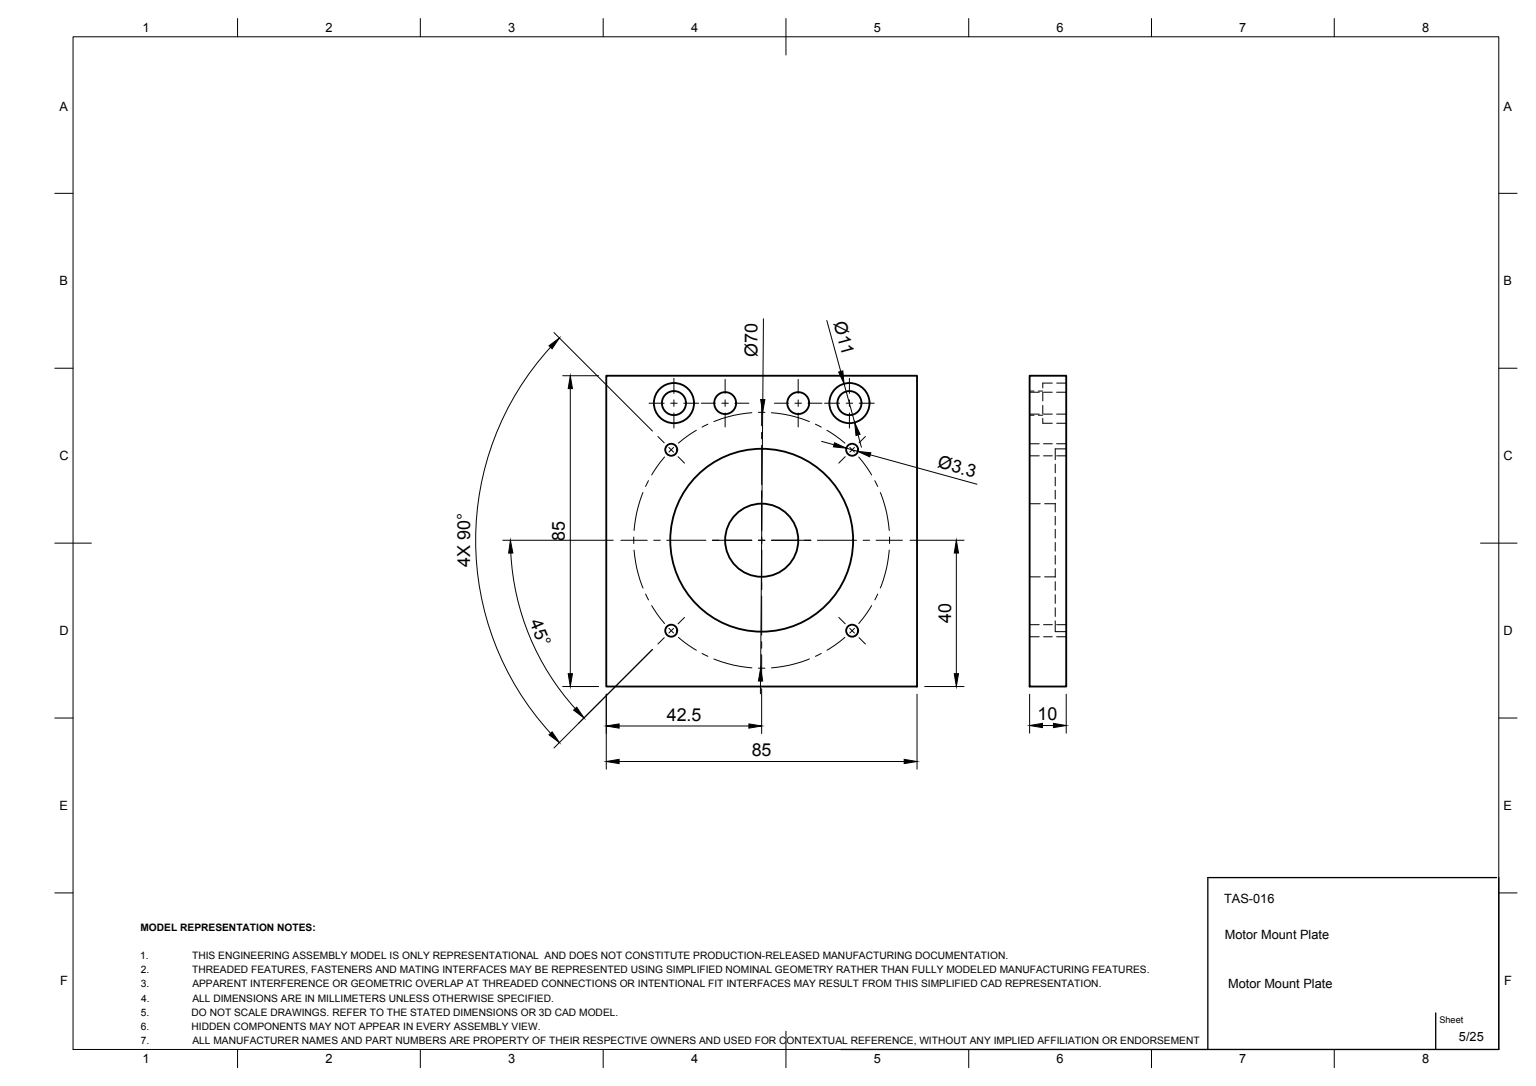
ISO-10303-21;
HEADER;
/* Generated by software containing ST-Developer
 * from STEP Tools, Inc. (www.steptools.com) 
 */

FILE_DESCRIPTION(
/* description */ ('STEP AP214'),
/* implementation_level */ '2;1');

FILE_NAME(
/* name */ 'Motor Mount Plate.step',
/* time_stamp */ '2026-11-15T14:55:55-08:00',
/* author */ (''),
/* organization */ (''),
/* preprocessor_version */ 'ST-DEVELOPER v20.2',
/* originating_system */ 'Autodesk Translation Framework v15.17.0.0',
/* authorisation */ '');

FILE_SCHEMA (('AUTOMOTIVE_DESIGN { 1 0 10303 214 3 1 1 }'));
ENDSEC;

DATA;
#10=MECHANICAL_DESIGN_GEOMETRIC_PRESENTATION_REPRESENTATION('',(#938),#57079);
#878=SHAPE_REPRESENTATION_RELATIONSHIP('SRR','None',#57264,#907);
#907=ADVANCED_BREP_SHAPE_REPRESENTATION('',(#975),#57056);
#938=STYLED_ITEM('',(#57444),#975);
#975=MANIFOLD_SOLID_BREP('Body1',#24538);
#1109=FACE_BOUND('',#3951,.T.);
#1110=FACE_BOUND('',#3952,.T.);
#1111=FACE_BOUND('',#3953,.T.);
#1112=FACE_BOUND('',#3954,.T.);
#1113=FACE_BOUND('',#3955,.T.);
#1114=FACE_BOUND('',#3956,.T.);
#1115=FACE_BOUND('',#3957,.T.);
#1116=FACE_BOUND('',#3958,.T.);
#1117=FACE_BOUND('',#3959,.T.);
#1118=FACE_BOUND('',#3965,.T.);
#1119=FACE_BOUND('',#3966,.T.);
#1120=FACE_BOUND('',#3967,.T.);
#1121=FACE_BOUND('',#3968,.T.);
#1122=FACE_BOUND('',#3969,.T.);
#1123=FACE_BOUND('',#3970,.T.);
#1124=FACE_BOUND('',#3971,.T.);
#1125=FACE_BOUND('',#3972,.T.);
#1126=FACE_BOUND('',#3973,.T.);
#1127=FACE_BOUND('',#3975,.T.);
#1128=FACE_BOUND('',#3977,.T.);
#1129=FACE_BOUND('',#3979,.T.);
#1524=PLANE('',#25459);
#1525=PLANE('',#25460);
#1526=PLANE('',#25461);
#1527=PLANE('',#25462);
#1528=PLANE('',#25463);
#1529=PLANE('',#25464);
#1530=PLANE('',#25465);
#1531=PLANE('',#25466);
#1532=PLANE('',#25467);
#2454=FACE_OUTER_BOUND('',#3938,.T.);
#2455=FACE_OUTER_BOUND('',#3939,.T.);
#2456=FACE_OUTER_BOUND('',#3940,.T.);
#2457=FACE_OUTER_BOUND('',#3941,.T.);
#2458=FACE_OUTER_BOUND('',#3942,.T.);
#2459=FACE_OUTER_BOUND('',#3943,.T.);
#2460=FACE_OUTER_BOUND('',#3944,.T.);
#2461=FACE_OUTER_BOUND('',#3945,.T.);
#2462=FACE_OUTER_BOUND('',#3946,.T.);
#2463=FACE_OUTER_BOUND('',#3947,.T.);
#2464=FACE_OUTER_BOUND('',#3948,.T.);
#2465=FACE_OUTER_BOUND('',#3949,.T.);
#2466=FACE_OUTER_BOUND('',#3950,.T.);
#2467=FACE_OUTER_BOUND('',#3960,.T.);
#2468=FACE_OUTER_BOUND('',#3961,.T.);
#2469=FACE_OUTER_BOUND('',#3962,.T.);
#2470=FACE_OUTER_BOUND('',#3963,.T.);
#2471=FACE_OUTER_BOUND('',#3964,.T.);
#2472=FACE_OUTER_BOUND('',#3974,.T.);
#2473=FACE_OUTER_BOUND('',#3976,.T.);
#2474=FACE_OUTER_BOUND('',#3978,.T.);
#3938=EDGE_LOOP('',(#17264,#17265,#17266,#17267));
#3939=EDGE_LOOP('',(#17268,#17269,#17270,#17271));
#3940=EDGE_LOOP('',(#17272,#17273,#17274,#17275));
#3941=EDGE_LOOP('',(#17276,#17277,#17278,#17279));
#3942=EDGE_LOOP('',(#17280,#17281,#17282,#17283));
#3943=EDGE_LOOP('',(#17284,#17285,#17286,#17287));
#3944=EDGE_LOOP('',(#17288,#17289,#17290,#17291));
#3945=EDGE_LOOP('',(#17292,#17293,#17294,#17295));
#3946=EDGE_LOOP('',(#17296,#17297,#17298,#17299));
#3947=EDGE_LOOP('',(#17300,#17301,#17302,#17303));
#3948=EDGE_LOOP('',(#17304,#17305,#17306,#17307));
#3949=EDGE_LOOP('',(#17308,#17309,#17310,#17311));
#3950=EDGE_LOOP('',(#17312,#17313,#17314,#17315));
#3951=EDGE_LOOP('',(#17316));
#3952=EDGE_LOOP('',(#17317));
#3953=EDGE_LOOP('',(#17318));
#3954=EDGE_LOOP('',(#17319));
#3955=EDGE_LOOP('',(#17320));
#3956=EDGE_LOOP('',(#17321));
#3957=EDGE_LOOP('',(#17322));
#3958=EDGE_LOOP('',(#17323));
#3959=EDGE_LOOP('',(#17324));
#3960=EDGE_LOOP('',(#17325,#17326,#17327,#17328));
#3961=EDGE_LOOP('',(#17329,#17330,#17331,#17332));
#3962=EDGE_LOOP('',(#17333,#17334,#17335,#17336));
#3963=EDGE_LOOP('',(#17337,#17338,#17339,#17340));
#3964=EDGE_LOOP('',(#17341,#17342,#17343,#17344));
#3965=EDGE_LOOP('',(#17345));
#3966=EDGE_LOOP('',(#17346));
#3967=EDGE_LOOP('',(#17347));
#3968=EDGE_LOOP('',(#17348));
#3969=EDGE_LOOP('',(#17349));
#3970=EDGE_LOOP('',(#17350));
#3971=EDGE_LOOP('',(#17351));
#3972=EDGE_LOOP('',(#17352));
#3973=EDGE_LOOP('',(#17353));
#3974=EDGE_LOOP('',(#17354));
#3975=EDGE_LOOP('',(#17355));
#3976=EDGE_LOOP('',(#17356));
#3977=EDGE_LOOP('',(#17357));
#3978=EDGE_LOOP('',(#17358));
#3979=EDGE_LOOP('',(#17359));
#5689=LINE('',#36296,#7656);
#5690=LINE('',#36302,#7657);
#5691=LINE('',#36308,#7658);
#5692=LINE('',#36314,#7659);
#5693=LINE('',#36320,#7660);
#5694=LINE('',#36326,#7661);
#5695=LINE('',#36332,#7662);
#5696=LINE('',#36338,#7663);
#5697=LINE('',#36344,#7664);
#5698=LINE('',#36350,#7665);
#5699=LINE('',#36356,#7666);
#5700=LINE('',#36362,#7667);
#5701=LINE('',#36367,#7668);
#5702=LINE('',#36369,#7669);
#5703=LINE('',#36371,#7670);
#5704=LINE('',#36372,#7671);
#5705=LINE('',#36376,#7672);
#5706=LINE('',#36377,#7673);
#5707=LINE('',#36378,#7674);
#5708=LINE('',#36381,#7675);
#5709=LINE('',#36382,#7676);
#5710=LINE('',#36385,#7677);
#5711=LINE('',#36386,#7678);
#5712=LINE('',#36388,#7679);
#7656=VECTOR('',#28999,1.65);
#7657=VECTOR('',#29006,1.65);
#7658=VECTOR('',#29013,1.65);
#7659=VECTOR('',#29020,1.65);
#7660=VECTOR('',#29027,3.);
#7661=VECTOR('',#29034,3.);
#7662=VECTOR('',#29041,5.5);
#7663=VECTOR('',#29048,3.3);
#7664=VECTOR('',#29055,5.5);
#7665=VECTOR('',#29062,3.3);
#7666=VECTOR('',#29069,10.);
#7667=VECTOR('',#29076,25.);
#7668=VECTOR('',#29081,1000.);
#7669=VECTOR('',#29082,1000.);
#7670=VECTOR('',#29083,1000.);
#7671=VECTOR('',#29084,1000.);
#7672=VECTOR('',#29087,1000.);
#7673=VECTOR('',#29088,1000.);
#7674=VECTOR('',#29089,1000.);
#7675=VECTOR('',#29092,1000.);
#7676=VECTOR('',#29093,1000.);
#7677=VECTOR('',#29096,1000.);
#7678=VECTOR('',#29097,1000.);
#7679=VECTOR('',#29100,1000.);
#9406=CIRCLE('',#25424,1.65);
#9407=CIRCLE('',#25425,1.65);
#9408=CIRCLE('',#25427,1.65);
#9409=CIRCLE('',#25428,1.65);
#9410=CIRCLE('',#25430,1.65);
#9411=CIRCLE('',#25431,1.65);
#9412=CIRCLE('',#25433,1.65);
#9413=CIRCLE('',#25434,1.65);
#9414=CIRCLE('',#25436,3.);
#9415=CIRCLE('',#25437,3.);
#9416=CIRCLE('',#25439,3.);
#9417=CIRCLE('',#25440,3.);
#9418=CIRCLE('',#25442,5.5);
#9419=CIRCLE('',#25443,5.5);
#9420=CIRCLE('',#25445,3.3);
#9421=CIRCLE('',#25446,3.3);
#9422=CIRCLE('',#25448,5.5);
#9423=CIRCLE('',#25449,5.5);
#9424=CIRCLE('',#25451,3.3);
#9425=CIRCLE('',#25452,3.3);
#9426=CIRCLE('',#25454,10.);
#9427=CIRCLE('',#25455,10.);
#9428=CIRCLE('',#25457,25.);
#9429=CIRCLE('',#25458,25.);
#10719=VERTEX_POINT('',#36293);
#10720=VERTEX_POINT('',#36295);
#10721=VERTEX_POINT('',#36299);
#10722=VERTEX_POINT('',#36301);
#10723=VERTEX_POINT('',#36305);
#10724=VERTEX_POINT('',#36307);
#10725=VERTEX_POINT('',#36311);
#10726=VERTEX_POINT('',#36313);
#10727=VERTEX_POINT('',#36317);
#10728=VERTEX_POINT('',#36319);
#10729=VERTEX_POINT('',#36323);
#10730=VERTEX_POINT('',#36325);
#10731=VERTEX_POINT('',#36329);
#10732=VERTEX_POINT('',#36331);
#10733=VERTEX_POINT('',#36335);
#10734=VERTEX_POINT('',#36337);
#10735=VERTEX_POINT('',#36341);
#10736=VERTEX_POINT('',#36343);
#10737=VERTEX_POINT('',#36347);
#10738=VERTEX_POINT('',#36349);
#10739=VERTEX_POINT('',#36353);
#10740=VERTEX_POINT('',#36355);
#10741=VERTEX_POINT('',#36359);
#10742=VERTEX_POINT('',#36361);
#10743=VERTEX_POINT('',#36365);
#10744=VERTEX_POINT('',#36366);
#10745=VERTEX_POINT('',#36368);
#10746=VERTEX_POINT('',#36370);
#10747=VERTEX_POINT('',#36374);
#10748=VERTEX_POINT('',#36375);
#10749=VERTEX_POINT('',#36380);
#10750=VERTEX_POINT('',#36384);
#13177=EDGE_CURVE('',#10719,#10719,#9406,.T.);
#13178=EDGE_CURVE('',#10719,#10720,#5689,.T.);
#13179=EDGE_CURVE('',#10720,#10720,#9407,.T.);
#13180=EDGE_CURVE('',#10721,#10721,#9408,.T.);
#13181=EDGE_CURVE('',#10721,#10722,#5690,.T.);
#13182=EDGE_CURVE('',#10722,#10722,#9409,.T.);
#13183=EDGE_CURVE('',#10723,#10723,#9410,.T.);
#13184=EDGE_CURVE('',#10723,#10724,#5691,.T.);
#13185=EDGE_CURVE('',#10724,#10724,#9411,.T.);
#13186=EDGE_CURVE('',#10725,#10725,#9412,.T.);
#13187=EDGE_CURVE('',#10725,#10726,#5692,.T.);
#13188=EDGE_CURVE('',#10726,#10726,#9413,.T.);
#13189=EDGE_CURVE('',#10727,#10727,#9414,.T.);
#13190=EDGE_CURVE('',#10727,#10728,#5693,.T.);
#13191=EDGE_CURVE('',#10728,#10728,#9415,.T.);
#13192=EDGE_CURVE('',#10729,#10729,#9416,.T.);
#13193=EDGE_CURVE('',#10729,#10730,#5694,.T.);
#13194=EDGE_CURVE('',#10730,#10730,#9417,.T.);
#13195=EDGE_CURVE('',#10731,#10731,#9418,.T.);
#13196=EDGE_CURVE('',#10731,#10732,#5695,.T.);
#13197=EDGE_CURVE('',#10732,#10732,#9419,.T.);
#13198=EDGE_CURVE('',#10733,#10733,#9420,.T.);
#13199=EDGE_CURVE('',#10733,#10734,#5696,.T.);
#13200=EDGE_CURVE('',#10734,#10734,#9421,.T.);
#13201=EDGE_CURVE('',#10735,#10735,#9422,.T.);
#13202=EDGE_CURVE('',#10735,#10736,#5697,.T.);
#13203=EDGE_CURVE('',#10736,#10736,#9423,.T.);
#13204=EDGE_CURVE('',#10737,#10737,#9424,.T.);
#13205=EDGE_CURVE('',#10737,#10738,#5698,.T.);
#13206=EDGE_CURVE('',#10738,#10738,#9425,.T.);
#13207=EDGE_CURVE('',#10739,#10739,#9426,.T.);
#13208=EDGE_CURVE('',#10739,#10740,#5699,.T.);
#13209=EDGE_CURVE('',#10740,#10740,#9427,.T.);
#13210=EDGE_CURVE('',#10741,#10741,#9428,.T.);
#13211=EDGE_CURVE('',#10741,#10742,#5700,.T.);
#13212=EDGE_CURVE('',#10742,#10742,#9429,.T.);
#13213=EDGE_CURVE('',#10743,#10744,#5701,.T.);
#13214=EDGE_CURVE('',#10744,#10745,#5702,.T.);
#13215=EDGE_CURVE('',#10745,#10746,#5703,.T.);
#13216=EDGE_CURVE('',#10746,#10743,#5704,.T.);
#13217=EDGE_CURVE('',#10747,#10748,#5705,.T.);
#13218=EDGE_CURVE('',#10744,#10748,#5706,.T.);
#13219=EDGE_CURVE('',#10743,#10747,#5707,.T.);
#13220=EDGE_CURVE('',#10748,#10749,#5708,.T.);
#13221=EDGE_CURVE('',#10745,#10749,#5709,.T.);
#13222=EDGE_CURVE('',#10749,#10750,#5710,.T.);
#13223=EDGE_CURVE('',#10746,#10750,#5711,.T.);
#13224=EDGE_CURVE('',#10750,#10747,#5712,.T.);
#17264=ORIENTED_EDGE('',*,*,#13177,.F.);
#17265=ORIENTED_EDGE('',*,*,#13178,.T.);
#17266=ORIENTED_EDGE('',*,*,#13179,.T.);
#17267=ORIENTED_EDGE('',*,*,#13178,.F.);
#17268=ORIENTED_EDGE('',*,*,#13180,.F.);
#17269=ORIENTED_EDGE('',*,*,#13181,.T.);
#17270=ORIENTED_EDGE('',*,*,#13182,.T.);
#17271=ORIENTED_EDGE('',*,*,#13181,.F.);
#17272=ORIENTED_EDGE('',*,*,#13183,.F.);
#17273=ORIENTED_EDGE('',*,*,#13184,.T.);
#17274=ORIENTED_EDGE('',*,*,#13185,.T.);
#17275=ORIENTED_EDGE('',*,*,#13184,.F.);
#17276=ORIENTED_EDGE('',*,*,#13186,.F.);
#17277=ORIENTED_EDGE('',*,*,#13187,.T.);
#17278=ORIENTED_EDGE('',*,*,#13188,.T.);
#17279=ORIENTED_EDGE('',*,*,#13187,.F.);
#17280=ORIENTED_EDGE('',*,*,#13189,.F.);
#17281=ORIENTED_EDGE('',*,*,#13190,.T.);
#17282=ORIENTED_EDGE('',*,*,#13191,.T.);
#17283=ORIENTED_EDGE('',*,*,#13190,.F.);
#17284=ORIENTED_EDGE('',*,*,#13192,.F.);
#17285=ORIENTED_EDGE('',*,*,#13193,.T.);
#17286=ORIENTED_EDGE('',*,*,#13194,.T.);
#17287=ORIENTED_EDGE('',*,*,#13193,.F.);
#17288=ORIENTED_EDGE('',*,*,#13195,.F.);
#17289=ORIENTED_EDGE('',*,*,#13196,.T.);
#17290=ORIENTED_EDGE('',*,*,#13197,.T.);
#17291=ORIENTED_EDGE('',*,*,#13196,.F.);
#17292=ORIENTED_EDGE('',*,*,#13198,.F.);
#17293=ORIENTED_EDGE('',*,*,#13199,.T.);
#17294=ORIENTED_EDGE('',*,*,#13200,.T.);
#17295=ORIENTED_EDGE('',*,*,#13199,.F.);
#17296=ORIENTED_EDGE('',*,*,#13201,.F.);
#17297=ORIENTED_EDGE('',*,*,#13202,.T.);
#17298=ORIENTED_EDGE('',*,*,#13203,.T.);
#17299=ORIENTED_EDGE('',*,*,#13202,.F.);
#17300=ORIENTED_EDGE('',*,*,#13204,.F.);
#17301=ORIENTED_EDGE('',*,*,#13205,.T.);
#17302=ORIENTED_EDGE('',*,*,#13206,.T.);
#17303=ORIENTED_EDGE('',*,*,#13205,.F.);
#17304=ORIENTED_EDGE('',*,*,#13207,.F.);
#17305=ORIENTED_EDGE('',*,*,#13208,.T.);
#17306=ORIENTED_EDGE('',*,*,#13209,.T.);
#17307=ORIENTED_EDGE('',*,*,#13208,.F.);
#17308=ORIENTED_EDGE('',*,*,#13210,.F.);
#17309=ORIENTED_EDGE('',*,*,#13211,.T.);
#17310=ORIENTED_EDGE('',*,*,#13212,.T.);
#17311=ORIENTED_EDGE('',*,*,#13211,.F.);
#17312=ORIENTED_EDGE('',*,*,#13213,.T.);
#17313=ORIENTED_EDGE('',*,*,#13214,.T.);
#17314=ORIENTED_EDGE('',*,*,#13215,.T.);
#17315=ORIENTED_EDGE('',*,*,#13216,.T.);
#17316=ORIENTED_EDGE('',*,*,#13185,.F.);
#17317=ORIENTED_EDGE('',*,*,#13179,.F.);
#17318=ORIENTED_EDGE('',*,*,#13182,.F.);
#17319=ORIENTED_EDGE('',*,*,#13188,.F.);
#17320=ORIENTED_EDGE('',*,*,#13191,.F.);
#17321=ORIENTED_EDGE('',*,*,#13194,.F.);
#17322=ORIENTED_EDGE('',*,*,#13197,.F.);
#17323=ORIENTED_EDGE('',*,*,#13203,.F.);
#17324=ORIENTED_EDGE('',*,*,#13212,.F.);
#17325=ORIENTED_EDGE('',*,*,#13217,.T.);
#17326=ORIENTED_EDGE('',*,*,#13218,.F.);
#17327=ORIENTED_EDGE('',*,*,#13213,.F.);
#17328=ORIENTED_EDGE('',*,*,#13219,.T.);
#17329=ORIENTED_EDGE('',*,*,#13220,.T.);
#17330=ORIENTED_EDGE('',*,*,#13221,.F.);
#17331=ORIENTED_EDGE('',*,*,#13214,.F.);
#17332=ORIENTED_EDGE('',*,*,#13218,.T.);
#17333=ORIENTED_EDGE('',*,*,#13222,.T.);
#17334=ORIENTED_EDGE('',*,*,#13223,.F.);
#17335=ORIENTED_EDGE('',*,*,#13215,.F.);
#17336=ORIENTED_EDGE('',*,*,#13221,.T.);
#17337=ORIENTED_EDGE('',*,*,#13224,.T.);
#17338=ORIENTED_EDGE('',*,*,#13219,.F.);
#17339=ORIENTED_EDGE('',*,*,#13216,.F.);
#17340=ORIENTED_EDGE('',*,*,#13223,.T.);
#17341=ORIENTED_EDGE('',*,*,#13217,.F.);
#17342=ORIENTED_EDGE('',*,*,#13224,.F.);
#17343=ORIENTED_EDGE('',*,*,#13222,.F.);
#17344=ORIENTED_EDGE('',*,*,#13220,.F.);
#17345=ORIENTED_EDGE('',*,*,#13177,.T.);
#17346=ORIENTED_EDGE('',*,*,#13180,.T.);
#17347=ORIENTED_EDGE('',*,*,#13183,.T.);
#17348=ORIENTED_EDGE('',*,*,#13186,.T.);
#17349=ORIENTED_EDGE('',*,*,#13189,.T.);
#17350=ORIENTED_EDGE('',*,*,#13192,.T.);
#17351=ORIENTED_EDGE('',*,*,#13198,.T.);
#17352=ORIENTED_EDGE('',*,*,#13204,.T.);
#17353=ORIENTED_EDGE('',*,*,#13207,.T.);
#17354=ORIENTED_EDGE('',*,*,#13210,.T.);
#17355=ORIENTED_EDGE('',*,*,#13209,.F.);
#17356=ORIENTED_EDGE('',*,*,#13201,.T.);
#17357=ORIENTED_EDGE('',*,*,#13206,.F.);
#17358=ORIENTED_EDGE('',*,*,#13195,.T.);
#17359=ORIENTED_EDGE('',*,*,#13200,.F.);
#22826=CYLINDRICAL_SURFACE('',#25423,1.65);
#22827=CYLINDRICAL_SURFACE('',#25426,1.65);
#22828=CYLINDRICAL_SURFACE('',#25429,1.65);
#22829=CYLINDRICAL_SURFACE('',#25432,1.65);
#22830=CYLINDRICAL_SURFACE('',#25435,3.);
#22831=CYLINDRICAL_SURFACE('',#25438,3.);
#22832=CYLINDRICAL_SURFACE('',#25441,5.5);
#22833=CYLINDRICAL_SURFACE('',#25444,3.3);
#22834=CYLINDRICAL_SURFACE('',#25447,5.5);
#22835=CYLINDRICAL_SURFACE('',#25450,3.3);
#22836=CYLINDRICAL_SURFACE('',#25453,10.);
#22837=CYLINDRICAL_SURFACE('',#25456,25.);
#23446=ADVANCED_FACE('',(#2454),#22826,.F.);
#23447=ADVANCED_FACE('',(#2455),#22827,.F.);
#23448=ADVANCED_FACE('',(#2456),#22828,.F.);
#23449=ADVANCED_FACE('',(#2457),#22829,.F.);
#23450=ADVANCED_FACE('',(#2458),#22830,.F.);
#23451=ADVANCED_FACE('',(#2459),#22831,.F.);
#23452=ADVANCED_FACE('',(#2460),#22832,.F.);
#23453=ADVANCED_FACE('',(#2461),#22833,.F.);
#23454=ADVANCED_FACE('',(#2462),#22834,.F.);
#23455=ADVANCED_FACE('',(#2463),#22835,.F.);
#23456=ADVANCED_FACE('',(#2464),#22836,.F.);
#23457=ADVANCED_FACE('',(#2465),#22837,.F.);
#23458=ADVANCED_FACE('',(#2466,#1109,#1110,#1111,#1112,#1113,#1114,#1115,
#1116,#1117),#1524,.F.);
#23459=ADVANCED_FACE('',(#2467),#1525,.F.);
#23460=ADVANCED_FACE('',(#2468),#1526,.F.);
#23461=ADVANCED_FACE('',(#2469),#1527,.F.);
#23462=ADVANCED_FACE('',(#2470),#1528,.F.);
#23463=ADVANCED_FACE('',(#2471,#1118,#1119,#1120,#1121,#1122,#1123,#1124,
#1125,#1126),#1529,.T.);
#23464=ADVANCED_FACE('',(#2472,#1127),#1530,.T.);
#23465=ADVANCED_FACE('',(#2473,#1128),#1531,.F.);
#23466=ADVANCED_FACE('',(#2474,#1129),#1532,.F.);
#24538=CLOSED_SHELL('',(#23446,#23447,#23448,#23449,#23450,#23451,#23452,
#23453,#23454,#23455,#23456,#23457,#23458,#23459,#23460,#23461,#23462,#23463,
#23464,#23465,#23466));
#25422=AXIS2_PLACEMENT_3D('',#36291,#28993,#28994);
#25423=AXIS2_PLACEMENT_3D('',#36292,#28995,#28996);
#25424=AXIS2_PLACEMENT_3D('',#36294,#28997,#28998);
#25425=AXIS2_PLACEMENT_3D('',#36297,#29000,#29001);
#25426=AXIS2_PLACEMENT_3D('',#36298,#29002,#29003);
#25427=AXIS2_PLACEMENT_3D('',#36300,#29004,#29005);
#25428=AXIS2_PLACEMENT_3D('',#36303,#29007,#29008);
#25429=AXIS2_PLACEMENT_3D('',#36304,#29009,#29010);
#25430=AXIS2_PLACEMENT_3D('',#36306,#29011,#29012);
#25431=AXIS2_PLACEMENT_3D('',#36309,#29014,#29015);
#25432=AXIS2_PLACEMENT_3D('',#36310,#29016,#29017);
#25433=AXIS2_PLACEMENT_3D('',#36312,#29018,#29019);
#25434=AXIS2_PLACEMENT_3D('',#36315,#29021,#29022);
#25435=AXIS2_PLACEMENT_3D('',#36316,#29023,#29024);
#25436=AXIS2_PLACEMENT_3D('',#36318,#29025,#29026);
#25437=AXIS2_PLACEMENT_3D('',#36321,#29028,#29029);
#25438=AXIS2_PLACEMENT_3D('',#36322,#29030,#29031);
#25439=AXIS2_PLACEMENT_3D('',#36324,#29032,#29033);
#25440=AXIS2_PLACEMENT_3D('',#36327,#29035,#29036);
#25441=AXIS2_PLACEMENT_3D('',#36328,#29037,#29038);
#25442=AXIS2_PLACEMENT_3D('',#36330,#29039,#29040);
#25443=AXIS2_PLACEMENT_3D('',#36333,#29042,#29043);
#25444=AXIS2_PLACEMENT_3D('',#36334,#29044,#29045);
#25445=AXIS2_PLACEMENT_3D('',#36336,#29046,#29047);
#25446=AXIS2_PLACEMENT_3D('',#36339,#29049,#29050);
#25447=AXIS2_PLACEMENT_3D('',#36340,#29051,#29052);
#25448=AXIS2_PLACEMENT_3D('',#36342,#29053,#29054);
#25449=AXIS2_PLACEMENT_3D('',#36345,#29056,#29057);
#25450=AXIS2_PLACEMENT_3D('',#36346,#29058,#29059);
#25451=AXIS2_PLACEMENT_3D('',#36348,#29060,#29061);
#25452=AXIS2_PLACEMENT_3D('',#36351,#29063,#29064);
#25453=AXIS2_PLACEMENT_3D('',#36352,#29065,#29066);
#25454=AXIS2_PLACEMENT_3D('',#36354,#29067,#29068);
#25455=AXIS2_PLACEMENT_3D('',#36357,#29070,#29071);
#25456=AXIS2_PLACEMENT_3D('',#36358,#29072,#29073);
#25457=AXIS2_PLACEMENT_3D('',#36360,#29074,#29075);
#25458=AXIS2_PLACEMENT_3D('',#36363,#29077,#29078);
#25459=AXIS2_PLACEMENT_3D('',#36364,#29079,#29080);
#25460=AXIS2_PLACEMENT_3D('',#36373,#29085,#29086);
#25461=AXIS2_PLACEMENT_3D('',#36379,#29090,#29091);
#25462=AXIS2_PLACEMENT_3D('',#36383,#29094,#29095);
#25463=AXIS2_PLACEMENT_3D('',#36387,#29098,#29099);
#25464=AXIS2_PLACEMENT_3D('',#36389,#29101,#29102);
#25465=AXIS2_PLACEMENT_3D('',#36390,#29103,#29104);
#25466=AXIS2_PLACEMENT_3D('',#36391,#29105,#29106);
#25467=AXIS2_PLACEMENT_3D('',#36392,#29107,#29108);
#28993=DIRECTION('axis',(0.,0.,1.));
#28994=DIRECTION('refdir',(1.,0.,0.));
#28995=DIRECTION('center_axis',(0.,0.,1.));
#28996=DIRECTION('ref_axis',(1.,0.,0.));
#28997=DIRECTION('center_axis',(0.,0.,1.));
#28998=DIRECTION('ref_axis',(1.,0.,0.));
#28999=DIRECTION('',(0.,0.,1.));
#29000=DIRECTION('center_axis',(0.,0.,1.));
#29001=DIRECTION('ref_axis',(1.,0.,0.));
#29002=DIRECTION('center_axis',(0.,0.,1.));
#29003=DIRECTION('ref_axis',(1.,0.,0.));
#29004=DIRECTION('center_axis',(0.,0.,1.));
#29005=DIRECTION('ref_axis',(1.,0.,0.));
#29006=DIRECTION('',(0.,0.,1.));
#29007=DIRECTION('center_axis',(0.,0.,1.));
#29008=DIRECTION('ref_axis',(1.,0.,0.));
#29009=DIRECTION('center_axis',(0.,0.,1.));
#29010=DIRECTION('ref_axis',(1.,0.,0.));
#29011=DIRECTION('center_axis',(0.,0.,1.));
#29012=DIRECTION('ref_axis',(1.,0.,0.));
#29013=DIRECTION('',(0.,0.,1.));
#29014=DIRECTION('center_axis',(0.,0.,1.));
#29015=DIRECTION('ref_axis',(1.,0.,0.));
#29016=DIRECTION('center_axis',(0.,0.,1.));
#29017=DIRECTION('ref_axis',(1.,0.,0.));
#29018=DIRECTION('center_axis',(0.,0.,1.));
#29019=DIRECTION('ref_axis',(1.,0.,0.));
#29020=DIRECTION('',(0.,0.,1.));
#29021=DIRECTION('center_axis',(0.,0.,1.));
#29022=DIRECTION('ref_axis',(1.,0.,0.));
#29023=DIRECTION('center_axis',(0.,0.,1.));
#29024=DIRECTION('ref_axis',(1.,0.,0.));
#29025=DIRECTION('center_axis',(0.,0.,1.));
#29026=DIRECTION('ref_axis',(1.,0.,0.));
#29027=DIRECTION('',(0.,0.,1.));
#29028=DIRECTION('center_axis',(0.,0.,1.));
#29029=DIRECTION('ref_axis',(1.,0.,0.));
#29030=DIRECTION('center_axis',(0.,0.,1.));
#29031=DIRECTION('ref_axis',(1.,0.,0.));
#29032=DIRECTION('center_axis',(0.,0.,1.));
#29033=DIRECTION('ref_axis',(1.,0.,0.));
#29034=DIRECTION('',(0.,0.,1.));
#29035=DIRECTION('center_axis',(0.,0.,1.));
#29036=DIRECTION('ref_axis',(1.,0.,0.));
#29037=DIRECTION('center_axis',(0.,0.,1.));
#29038=DIRECTION('ref_axis',(1.,0.,0.));
#29039=DIRECTION('center_axis',(0.,0.,1.));
#29040=DIRECTION('ref_axis',(1.,0.,0.));
#29041=DIRECTION('',(0.,0.,1.));
#29042=DIRECTION('center_axis',(0.,0.,1.));
#29043=DIRECTION('ref_axis',(1.,0.,0.));
#29044=DIRECTION('center_axis',(0.,0.,1.));
#29045=DIRECTION('ref_axis',(1.,0.,0.));
#29046=DIRECTION('center_axis',(0.,0.,1.));
#29047=DIRECTION('ref_axis',(1.,0.,0.));
#29048=DIRECTION('',(0.,0.,1.));
#29049=DIRECTION('center_axis',(0.,0.,1.));
#29050=DIRECTION('ref_axis',(1.,0.,0.));
#29051=DIRECTION('center_axis',(0.,0.,1.));
#29052=DIRECTION('ref_axis',(1.,0.,0.));
#29053=DIRECTION('center_axis',(0.,0.,1.));
#29054=DIRECTION('ref_axis',(1.,0.,0.));
#29055=DIRECTION('',(0.,0.,1.));
#29056=DIRECTION('center_axis',(0.,0.,1.));
#29057=DIRECTION('ref_axis',(1.,0.,0.));
#29058=DIRECTION('center_axis',(0.,0.,1.));
#29059=DIRECTION('ref_axis',(1.,0.,0.));
#29060=DIRECTION('center_axis',(0.,0.,1.));
#29061=DIRECTION('ref_axis',(1.,0.,0.));
#29062=DIRECTION('',(0.,0.,1.));
#29063=DIRECTION('center_axis',(0.,0.,1.));
#29064=DIRECTION('ref_axis',(1.,0.,0.));
#29065=DIRECTION('center_axis',(0.,0.,1.));
#29066=DIRECTION('ref_axis',(1.,0.,0.));
#29067=DIRECTION('center_axis',(0.,0.,1.));
#29068=DIRECTION('ref_axis',(1.,0.,0.));
#29069=DIRECTION('',(0.,0.,1.));
#29070=DIRECTION('center_axis',(0.,0.,1.));
#29071=DIRECTION('ref_axis',(1.,0.,0.));
#29072=DIRECTION('center_axis',(0.,0.,1.));
#29073=DIRECTION('ref_axis',(1.,0.,0.));
#29074=DIRECTION('center_axis',(0.,0.,1.));
#29075=DIRECTION('ref_axis',(1.,0.,0.));
#29076=DIRECTION('',(0.,0.,1.));
#29077=DIRECTION('center_axis',(0.,0.,1.));
#29078=DIRECTION('ref_axis',(1.,0.,0.));
#29079=DIRECTION('center_axis',(0.,0.,-1.));
#29080=DIRECTION('ref_axis',(-1.,0.,0.));
#29081=DIRECTION('',(0.,1.,0.));
#29082=DIRECTION('',(-1.,0.,0.));
#29083=DIRECTION('',(0.,-1.,0.));
#29084=DIRECTION('',(1.,0.,0.));
#29085=DIRECTION('center_axis',(-1.,0.,0.));
#29086=DIRECTION('ref_axis',(0.,0.,1.));
#29087=DIRECTION('',(0.,1.,0.));
#29088=DIRECTION('',(0.,0.,-1.));
#29089=DIRECTION('',(0.,0.,-1.));
#29090=DIRECTION('center_axis',(0.,-1.,0.));
#29091=DIRECTION('ref_axis',(0.,0.,-1.));
#29092=DIRECTION('',(-1.,0.,0.));
#29093=DIRECTION('',(0.,0.,-1.));
#29094=DIRECTION('center_axis',(1.,0.,0.));
#29095=DIRECTION('ref_axis',(0.,0.,-1.));
#29096=DIRECTION('',(0.,-1.,0.));
#29097=DIRECTION('',(0.,0.,-1.));
#29098=DIRECTION('center_axis',(0.,1.,0.));
#29099=DIRECTION('ref_axis',(0.,0.,1.));
#29100=DIRECTION('',(1.,0.,0.));
#29101=DIRECTION('center_axis',(0.,0.,-1.));
#29102=DIRECTION('ref_axis',(-1.,0.,0.));
#29103=DIRECTION('center_axis',(0.,0.,1.));
#29104=DIRECTION('ref_axis',(1.,0.,0.));
#29105=DIRECTION('center_axis',(0.,0.,-1.));
#29106=DIRECTION('ref_axis',(-1.,0.,0.));
#29107=DIRECTION('center_axis',(0.,0.,-1.));
#29108=DIRECTION('ref_axis',(-1.,0.,0.));
#36291=CARTESIAN_POINT('',(0.,0.,0.));
#36292=CARTESIAN_POINT('Origin',(-24.7487373415288,22.2487373415298,5.));
#36293=CARTESIAN_POINT('',(-26.3987373415288,22.2487373415298,-5.));
#36294=CARTESIAN_POINT('Origin',(-24.7487373415288,22.2487373415298,-5.));
#36295=CARTESIAN_POINT('',(-26.3987373415288,22.2487373415298,5.));
#36296=CARTESIAN_POINT('',(-26.3987373415288,22.2487373415298,5.));
#36297=CARTESIAN_POINT('Origin',(-24.7487373415288,22.2487373415298,5.));
#36298=CARTESIAN_POINT('Origin',(-24.7487373415293,-27.2487373415288,5.));
#36299=CARTESIAN_POINT('',(-26.3987373415293,-27.2487373415288,-5.));
#36300=CARTESIAN_POINT('Origin',(-24.7487373415293,-27.2487373415288,-5.));
#36301=CARTESIAN_POINT('',(-26.3987373415293,-27.2487373415288,5.));
#36302=CARTESIAN_POINT('',(-26.3987373415293,-27.2487373415288,5.));
#36303=CARTESIAN_POINT('Origin',(-24.7487373415293,-27.2487373415288,5.));
#36304=CARTESIAN_POINT('Origin',(24.7487373415289,-27.2487373415291,5.));
#36305=CARTESIAN_POINT('',(23.0987373415289,-27.2487373415291,-5.));
#36306=CARTESIAN_POINT('Origin',(24.7487373415289,-27.2487373415291,-5.));
#36307=CARTESIAN_POINT('',(23.0987373415289,-27.2487373415291,5.));
#36308=CARTESIAN_POINT('',(23.0987373415289,-27.2487373415291,5.));
#36309=CARTESIAN_POINT('Origin',(24.7487373415289,-27.2487373415291,5.));
#36310=CARTESIAN_POINT('Origin',(24.7487373415293,22.2487373415293,5.));
#36311=CARTESIAN_POINT('',(23.0987373415293,22.2487373415293,-5.));
#36312=CARTESIAN_POINT('Origin',(24.7487373415293,22.2487373415293,-5.));
#36313=CARTESIAN_POINT('',(23.0987373415293,22.2487373415293,5.));
#36314=CARTESIAN_POINT('',(23.0987373415293,22.2487373415293,5.));
#36315=CARTESIAN_POINT('Origin',(24.7487373415293,22.2487373415293,5.));
#36316=CARTESIAN_POINT('Origin',(-10.,35.,5.));
#36317=CARTESIAN_POINT('',(-13.,35.,-5.));
#36318=CARTESIAN_POINT('Origin',(-10.,35.,-5.));
#36319=CARTESIAN_POINT('',(-13.,35.,5.));
#36320=CARTESIAN_POINT('',(-13.,35.,5.));
#36321=CARTESIAN_POINT('Origin',(-10.,35.,5.));
#36322=CARTESIAN_POINT('Origin',(10.,35.,5.));
#36323=CARTESIAN_POINT('',(7.,35.,-5.));
#36324=CARTESIAN_POINT('Origin',(10.,35.,-5.));
#36325=CARTESIAN_POINT('',(7.,35.,5.));
#36326=CARTESIAN_POINT('',(7.,35.,5.));
#36327=CARTESIAN_POINT('Origin',(10.,35.,5.));
#36328=CARTESIAN_POINT('Origin',(-24.,35.,5.));
#36329=CARTESIAN_POINT('',(-29.5,35.,-1.4));
#36330=CARTESIAN_POINT('Origin',(-24.,35.,-1.4));
#36331=CARTESIAN_POINT('',(-29.5,35.,5.));
#36332=CARTESIAN_POINT('',(-29.5,35.,5.));
#36333=CARTESIAN_POINT('Origin',(-24.,35.,5.));
#36334=CARTESIAN_POINT('Origin',(-24.,35.,5.));
#36335=CARTESIAN_POINT('',(-27.3,35.,-5.));
#36336=CARTESIAN_POINT('Origin',(-24.,35.,-5.));
#36337=CARTESIAN_POINT('',(-27.3,35.,-1.4));
#36338=CARTESIAN_POINT('',(-27.3,35.,5.));
#36339=CARTESIAN_POINT('Origin',(-24.,35.,-1.4));
#36340=CARTESIAN_POINT('Origin',(24.,35.,5.));
#36341=CARTESIAN_POINT('',(18.5,35.,-1.4));
#36342=CARTESIAN_POINT('Origin',(24.,35.,-1.4));
#36343=CARTESIAN_POINT('',(18.5,35.,5.));
#36344=CARTESIAN_POINT('',(18.5,35.,5.));
#36345=CARTESIAN_POINT('Origin',(24.,35.,5.));
#36346=CARTESIAN_POINT('Origin',(24.,35.,5.));
#36347=CARTESIAN_POINT('',(20.7,35.,-5.));
#36348=CARTESIAN_POINT('Origin',(24.,35.,-5.));
#36349=CARTESIAN_POINT('',(20.7,35.,-1.4));
#36350=CARTESIAN_POINT('',(20.7,35.,5.));
#36351=CARTESIAN_POINT('Origin',(24.,35.,-1.4));
#36352=CARTESIAN_POINT('Origin',(-1.20882209737476E-14,-2.49999999999972,
-5.));
#36353=CARTESIAN_POINT('',(-10.,-2.49999999999972,-5.));
#36354=CARTESIAN_POINT('Origin',(-1.20882209737476E-14,-2.49999999999972,
-5.));
#36355=CARTESIAN_POINT('',(-10.,-2.49999999999972,2.));
#36356=CARTESIAN_POINT('',(-10.,-2.49999999999972,-5.));
#36357=CARTESIAN_POINT('Origin',(-1.20882209737476E-14,-2.49999999999972,
2.));
#36358=CARTESIAN_POINT('Origin',(-1.20882209737476E-14,-2.49999999999972,
2.));
#36359=CARTESIAN_POINT('',(-25.,-2.49999999999972,2.));
#36360=CARTESIAN_POINT('Origin',(-1.20882209737476E-14,-2.49999999999972,
2.));
#36361=CARTESIAN_POINT('',(-25.,-2.49999999999972,5.));
#36362=CARTESIAN_POINT('',(-25.,-2.49999999999972,2.));
#36363=CARTESIAN_POINT('Origin',(-1.20882209737476E-14,-2.49999999999972,
5.));
#36364=CARTESIAN_POINT('Origin',(0.,0.,5.));
#36365=CARTESIAN_POINT('',(42.5,-42.5,5.));
#36366=CARTESIAN_POINT('',(42.5,42.5,5.));
#36367=CARTESIAN_POINT('',(42.5,-42.5,5.));
#36368=CARTESIAN_POINT('',(-42.5,42.5,5.));
#36369=CARTESIAN_POINT('',(-42.5,42.5,5.));
#36370=CARTESIAN_POINT('',(-42.5,-42.5,5.));
#36371=CARTESIAN_POINT('',(-42.5,-42.5,5.));
#36372=CARTESIAN_POINT('',(-42.5,-42.5,5.));
#36373=CARTESIAN_POINT('Origin',(42.5,-42.5,5.));
#36374=CARTESIAN_POINT('',(42.5,-42.5,-5.));
#36375=CARTESIAN_POINT('',(42.5,42.5,-5.));
#36376=CARTESIAN_POINT('',(42.5,-42.5,-5.));
#36377=CARTESIAN_POINT('',(42.5,42.5,5.));
#36378=CARTESIAN_POINT('',(42.5,-42.5,5.));
#36379=CARTESIAN_POINT('Origin',(-42.5,42.5,5.));
#36380=CARTESIAN_POINT('',(-42.5,42.5,-5.));
#36381=CARTESIAN_POINT('',(-42.5,42.5,-5.));
#36382=CARTESIAN_POINT('',(-42.5,42.5,5.));
#36383=CARTESIAN_POINT('Origin',(-42.5,-42.5,5.));
#36384=CARTESIAN_POINT('',(-42.5,-42.5,-5.));
#36385=CARTESIAN_POINT('',(-42.5,-42.5,-5.));
#36386=CARTESIAN_POINT('',(-42.5,-42.5,5.));
#36387=CARTESIAN_POINT('Origin',(-42.5,-42.5,5.));
#36388=CARTESIAN_POINT('',(-42.5,-42.5,-5.));
#36389=CARTESIAN_POINT('Origin',(0.,0.,-5.));
#36390=CARTESIAN_POINT('Origin',(-1.20882209737476E-14,-2.49999999999972,
2.));
#36391=CARTESIAN_POINT('Origin',(27.3,35.,-1.4));
#36392=CARTESIAN_POINT('Origin',(-20.7,35.,-1.4));
#57017=UNCERTAINTY_MEASURE_WITH_UNIT(LENGTH_MEASURE(0.01),#57080,
'DISTANCE_ACCURACY_VALUE',
'Maximum model space distance between geometric entities at asserted c
onnectivities');
#57040=UNCERTAINTY_MEASURE_WITH_UNIT(LENGTH_MEASURE(0.01),#57080,
'DISTANCE_ACCURACY_VALUE',
'Maximum model space distance between geometric entities at asserted c
onnectivities');
#57056=(
GEOMETRIC_REPRESENTATION_CONTEXT(3)
GLOBAL_UNCERTAINTY_ASSIGNED_CONTEXT((#57017))
GLOBAL_UNIT_ASSIGNED_CONTEXT((#57080,#57082,#57083))
REPRESENTATION_CONTEXT('','3D')
);
#57079=(
GEOMETRIC_REPRESENTATION_CONTEXT(3)
GLOBAL_UNCERTAINTY_ASSIGNED_CONTEXT((#57040))
GLOBAL_UNIT_ASSIGNED_CONTEXT((#57080,#57082,#57083))
REPRESENTATION_CONTEXT('','3D')
);
#57080=(
LENGTH_UNIT()
NAMED_UNIT(*)
SI_UNIT(.MILLI.,.METRE.)
);
#57082=(
NAMED_UNIT(*)
PLANE_ANGLE_UNIT()
SI_UNIT($,.RADIAN.)
);
#57083=(
NAMED_UNIT(*)
SI_UNIT($,.STERADIAN.)
SOLID_ANGLE_UNIT()
);
#57099=SHAPE_DEFINITION_REPRESENTATION(#57145,#57264);
#57145=PRODUCT_DEFINITION_SHAPE('',$,#57303);
#57264=SHAPE_REPRESENTATION('',(#25422),#57056);
#57287=PRODUCT_DEFINITION_CONTEXT('part definition',#57403,'design');
#57303=PRODUCT_DEFINITION('Motor Mount Plate','Motor Mount Plate',#57341,
#57287);
#57341=PRODUCT_DEFINITION_FORMATION('',$,#57420);
#57403=APPLICATION_CONTEXT(
'Core Data for Automotive Mechanical Design Process');
#57404=PRODUCT_CONTEXT('part definition',#57403,'mechanical');
#57420=PRODUCT('Motor Mount Plate','Motor Mount Plate',$,(#57404));
#57444=PRESENTATION_STYLE_ASSIGNMENT((#57446));
#57446=SURFACE_STYLE_USAGE(.BOTH.,#57448);
#57448=SURFACE_SIDE_STYLE('',(#57450));
#57450=SURFACE_STYLE_FILL_AREA(#57452);
#57452=FILL_AREA_STYLE('Opaque(202,209,238)',(#57454));
#57454=FILL_AREA_STYLE_COLOUR('Opaque(202,209,238)',#57456);
#57456=COLOUR_RGB('Opaque(202,209,238)',0.792156862745098,0.819607843137255,
0.933333333333333);
ENDSEC;
END-ISO-10303-21;
